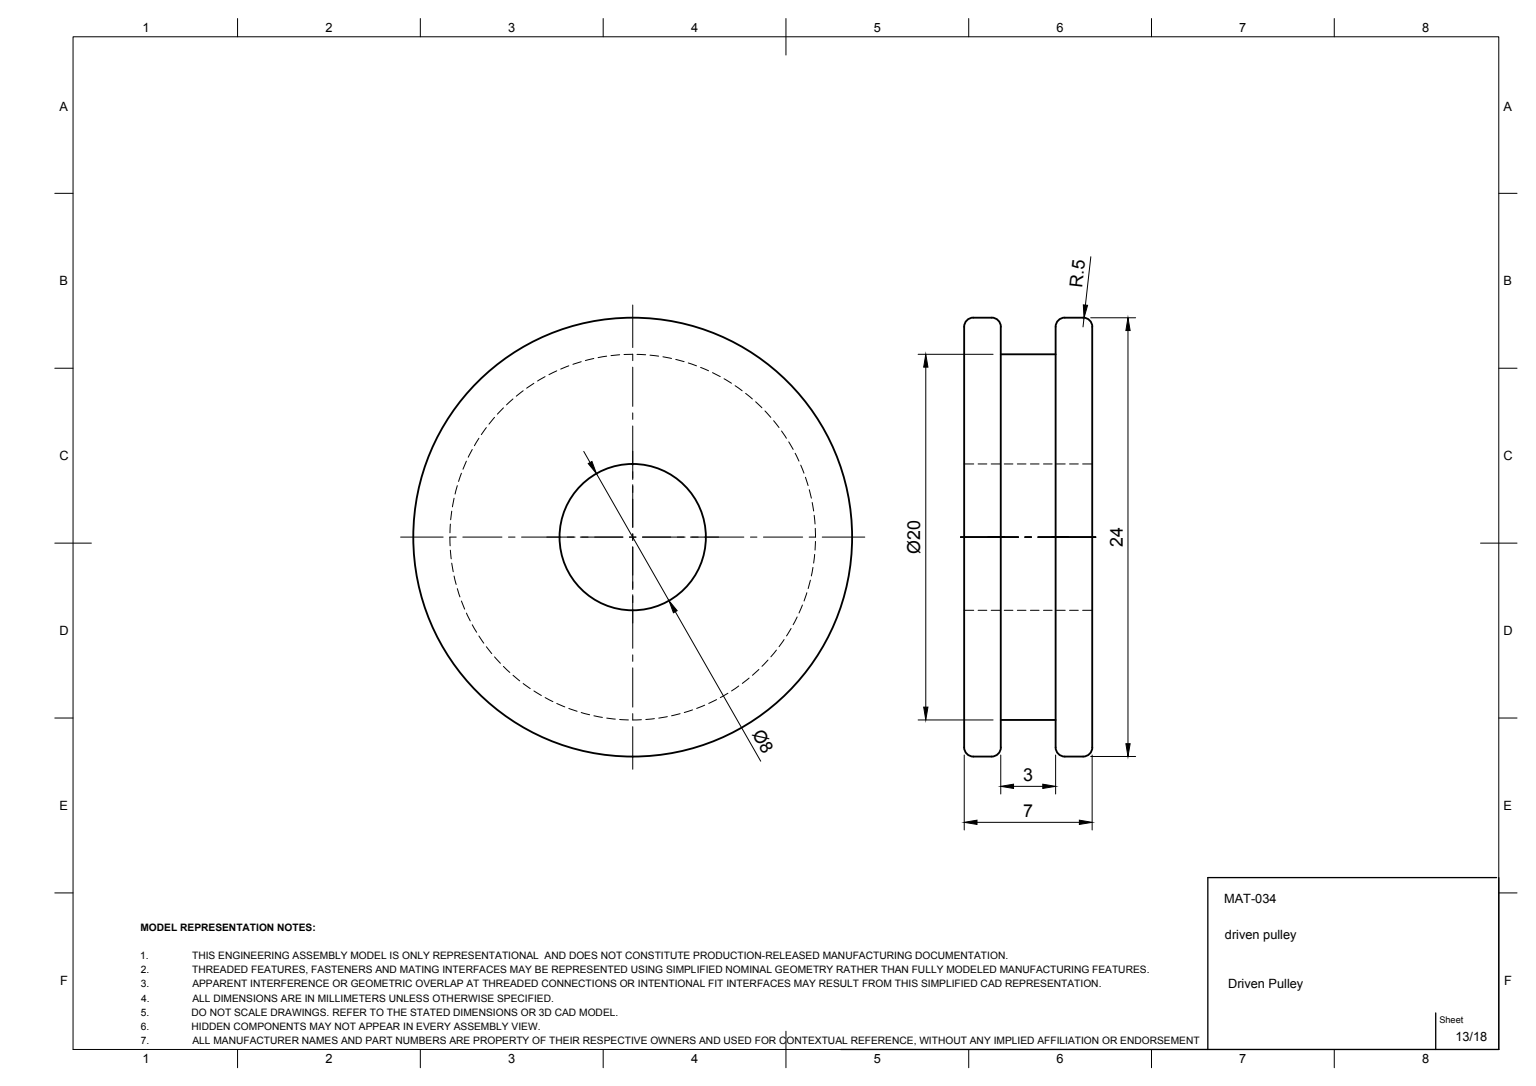
ISO-10303-21;
HEADER;
/* Generated by software containing ST-Developer
 * from STEP Tools, Inc. (www.steptools.com) 
 */

FILE_DESCRIPTION(
/* description */ ('STEP AP214'),
/* implementation_level */ '2;1');

FILE_NAME(
/* name */ 'Driven Pulley.step',
/* time_stamp */ '2026-11-14T09:24:36-08:00',
/* author */ (''),
/* organization */ (''),
/* preprocessor_version */ 'ST-DEVELOPER v20.2',
/* originating_system */ 'Autodesk Translation Framework v15.17.0.0',
/* authorisation */ '');

FILE_SCHEMA (('AUTOMOTIVE_DESIGN { 1 0 10303 214 3 1 1 }'));
ENDSEC;

DATA;
#10=MECHANICAL_DESIGN_GEOMETRIC_PRESENTATION_REPRESENTATION('',(#209),#18867);
#150=TOROIDAL_SURFACE('',#11551,11.5,0.5);
#151=TOROIDAL_SURFACE('',#11555,11.5,0.5);
#152=TOROIDAL_SURFACE('',#11560,11.5,0.5);
#153=TOROIDAL_SURFACE('',#11564,11.5,0.5);
#177=SHAPE_REPRESENTATION_RELATIONSHIP('SRR','None',#18941,#193);
#193=ADVANCED_BREP_SHAPE_REPRESENTATION('',(#233),#18857);
#209=STYLED_ITEM('',(#19027),#233);
#233=MANIFOLD_SOLID_BREP('Body1',#10964);
#323=FACE_BOUND('',#1619,.T.);
#324=FACE_BOUND('',#1621,.T.);
#325=FACE_BOUND('',#1623,.T.);
#326=FACE_BOUND('',#1625,.T.);
#519=PLANE('',#11574);
#520=PLANE('',#11575);
#521=PLANE('',#11576);
#522=PLANE('',#11577);
#942=FACE_OUTER_BOUND('',#1610,.T.);
#943=FACE_OUTER_BOUND('',#1611,.T.);
#944=FACE_OUTER_BOUND('',#1612,.T.);
#945=FACE_OUTER_BOUND('',#1613,.T.);
#946=FACE_OUTER_BOUND('',#1614,.T.);
#947=FACE_OUTER_BOUND('',#1615,.T.);
#948=FACE_OUTER_BOUND('',#1616,.T.);
#949=FACE_OUTER_BOUND('',#1617,.T.);
#950=FACE_OUTER_BOUND('',#1618,.T.);
#951=FACE_OUTER_BOUND('',#1620,.T.);
#952=FACE_OUTER_BOUND('',#1622,.T.);
#953=FACE_OUTER_BOUND('',#1624,.T.);
#1610=EDGE_LOOP('',(#8182,#8183,#8184,#8185));
#1611=EDGE_LOOP('',(#8186,#8187,#8188,#8189));
#1612=EDGE_LOOP('',(#8190,#8191,#8192,#8193,#8194));
#1613=EDGE_LOOP('',(#8195,#8196,#8197,#8198));
#1614=EDGE_LOOP('',(#8199,#8200,#8201,#8202,#8203));
#1615=EDGE_LOOP('',(#8204,#8205,#8206,#8207,#8208));
#1616=EDGE_LOOP('',(#8209,#8210,#8211,#8212));
#1617=EDGE_LOOP('',(#8213,#8214,#8215,#8216,#8217));
#1618=EDGE_LOOP('',(#8218));
#1619=EDGE_LOOP('',(#8219));
#1620=EDGE_LOOP('',(#8220));
#1621=EDGE_LOOP('',(#8221));
#1622=EDGE_LOOP('',(#8222));
#1623=EDGE_LOOP('',(#8223));
#1624=EDGE_LOOP('',(#8224));
#1625=EDGE_LOOP('',(#8225));
#2420=LINE('',#16727,#3434);
#2421=LINE('',#16758,#3435);
#2422=LINE('',#16763,#3436);
#2423=LINE('',#16766,#3437);
#3434=VECTOR('',#13458,4.);
#3435=VECTOR('',#13499,12.);
#3436=VECTOR('',#13504,10.);
#3437=VECTOR('',#13509,12.);
#4235=CIRCLE('',#11549,4.);
#4236=CIRCLE('',#11550,4.);
#4237=CIRCLE('',#11552,12.);
#4238=CIRCLE('',#11553,0.5);
#4239=CIRCLE('',#11554,11.5);
#4240=CIRCLE('',#11556,12.);
#4241=CIRCLE('',#11557,12.);
#4242=CIRCLE('',#11558,0.5);
#4243=CIRCLE('',#11559,11.5);
#4244=CIRCLE('',#11561,12.);
#4245=CIRCLE('',#11562,0.5);
#4246=CIRCLE('',#11563,11.5);
#4247=CIRCLE('',#11565,12.);
#4248=CIRCLE('',#11566,12.);
#4249=CIRCLE('',#11567,0.5);
#4250=CIRCLE('',#11568,11.5);
#4251=CIRCLE('',#11571,10.);
#4252=CIRCLE('',#11572,10.);
#4930=VERTEX_POINT('',#16724);
#4931=VERTEX_POINT('',#16726);
#4932=VERTEX_POINT('',#16730);
#4933=VERTEX_POINT('',#16732);
#4934=VERTEX_POINT('',#16736);
#4935=VERTEX_POINT('',#16737);
#4936=VERTEX_POINT('',#16740);
#4937=VERTEX_POINT('',#16744);
#4938=VERTEX_POINT('',#16746);
#4939=VERTEX_POINT('',#16750);
#4940=VERTEX_POINT('',#16751);
#4941=VERTEX_POINT('',#16754);
#4942=VERTEX_POINT('',#16760);
#4943=VERTEX_POINT('',#16762);
#6124=EDGE_CURVE('',#4930,#4930,#4235,.T.);
#6125=EDGE_CURVE('',#4930,#4931,#2420,.T.);
#6126=EDGE_CURVE('',#4931,#4931,#4236,.T.);
#6127=EDGE_CURVE('',#4932,#4932,#4237,.T.);
#6128=EDGE_CURVE('',#4932,#4933,#4238,.T.);
#6129=EDGE_CURVE('',#4933,#4933,#4239,.T.);
#6130=EDGE_CURVE('',#4934,#4935,#4240,.T.);
#6131=EDGE_CURVE('',#4935,#4934,#4241,.T.);
#6132=EDGE_CURVE('',#4935,#4936,#4242,.T.);
#6133=EDGE_CURVE('',#4936,#4936,#4243,.T.);
#6134=EDGE_CURVE('',#4937,#4937,#4244,.T.);
#6135=EDGE_CURVE('',#4937,#4938,#4245,.T.);
#6136=EDGE_CURVE('',#4938,#4938,#4246,.T.);
#6137=EDGE_CURVE('',#4939,#4940,#4247,.T.);
#6138=EDGE_CURVE('',#4940,#4939,#4248,.T.);
#6139=EDGE_CURVE('',#4940,#4941,#4249,.T.);
#6140=EDGE_CURVE('',#4941,#4941,#4250,.T.);
#6141=EDGE_CURVE('',#4934,#4932,#2421,.T.);
#6142=EDGE_CURVE('',#4942,#4942,#4251,.T.);
#6143=EDGE_CURVE('',#4942,#4943,#2422,.T.);
#6144=EDGE_CURVE('',#4943,#4943,#4252,.T.);
#6145=EDGE_CURVE('',#4939,#4937,#2423,.T.);
#8182=ORIENTED_EDGE('',*,*,#6124,.F.);
#8183=ORIENTED_EDGE('',*,*,#6125,.T.);
#8184=ORIENTED_EDGE('',*,*,#6126,.T.);
#8185=ORIENTED_EDGE('',*,*,#6125,.F.);
#8186=ORIENTED_EDGE('',*,*,#6127,.F.);
#8187=ORIENTED_EDGE('',*,*,#6128,.T.);
#8188=ORIENTED_EDGE('',*,*,#6129,.F.);
#8189=ORIENTED_EDGE('',*,*,#6128,.F.);
#8190=ORIENTED_EDGE('',*,*,#6130,.F.);
#8191=ORIENTED_EDGE('',*,*,#6131,.F.);
#8192=ORIENTED_EDGE('',*,*,#6132,.T.);
#8193=ORIENTED_EDGE('',*,*,#6133,.F.);
#8194=ORIENTED_EDGE('',*,*,#6132,.F.);
#8195=ORIENTED_EDGE('',*,*,#6134,.F.);
#8196=ORIENTED_EDGE('',*,*,#6135,.T.);
#8197=ORIENTED_EDGE('',*,*,#6136,.F.);
#8198=ORIENTED_EDGE('',*,*,#6135,.F.);
#8199=ORIENTED_EDGE('',*,*,#6137,.F.);
#8200=ORIENTED_EDGE('',*,*,#6138,.F.);
#8201=ORIENTED_EDGE('',*,*,#6139,.T.);
#8202=ORIENTED_EDGE('',*,*,#6140,.F.);
#8203=ORIENTED_EDGE('',*,*,#6139,.F.);
#8204=ORIENTED_EDGE('',*,*,#6130,.T.);
#8205=ORIENTED_EDGE('',*,*,#6131,.T.);
#8206=ORIENTED_EDGE('',*,*,#6141,.T.);
#8207=ORIENTED_EDGE('',*,*,#6127,.T.);
#8208=ORIENTED_EDGE('',*,*,#6141,.F.);
#8209=ORIENTED_EDGE('',*,*,#6142,.F.);
#8210=ORIENTED_EDGE('',*,*,#6143,.T.);
#8211=ORIENTED_EDGE('',*,*,#6144,.T.);
#8212=ORIENTED_EDGE('',*,*,#6143,.F.);
#8213=ORIENTED_EDGE('',*,*,#6137,.T.);
#8214=ORIENTED_EDGE('',*,*,#6138,.T.);
#8215=ORIENTED_EDGE('',*,*,#6145,.T.);
#8216=ORIENTED_EDGE('',*,*,#6134,.T.);
#8217=ORIENTED_EDGE('',*,*,#6145,.F.);
#8218=ORIENTED_EDGE('',*,*,#6129,.T.);
#8219=ORIENTED_EDGE('',*,*,#6124,.T.);
#8220=ORIENTED_EDGE('',*,*,#6140,.T.);
#8221=ORIENTED_EDGE('',*,*,#6126,.F.);
#8222=ORIENTED_EDGE('',*,*,#6136,.T.);
#8223=ORIENTED_EDGE('',*,*,#6142,.T.);
#8224=ORIENTED_EDGE('',*,*,#6133,.T.);
#8225=ORIENTED_EDGE('',*,*,#6144,.F.);
#10225=CYLINDRICAL_SURFACE('',#11548,4.);
#10226=CYLINDRICAL_SURFACE('',#11569,12.);
#10227=CYLINDRICAL_SURFACE('',#11570,10.);
#10228=CYLINDRICAL_SURFACE('',#11573,12.);
#10579=ADVANCED_FACE('',(#942),#10225,.F.);
#10580=ADVANCED_FACE('',(#943),#150,.T.);
#10581=ADVANCED_FACE('',(#944),#151,.T.);
#10582=ADVANCED_FACE('',(#945),#152,.T.);
#10583=ADVANCED_FACE('',(#946),#153,.T.);
#10584=ADVANCED_FACE('',(#947),#10226,.T.);
#10585=ADVANCED_FACE('',(#948),#10227,.T.);
#10586=ADVANCED_FACE('',(#949),#10228,.T.);
#10587=ADVANCED_FACE('',(#950,#323),#519,.F.);
#10588=ADVANCED_FACE('',(#951,#324),#520,.F.);
#10589=ADVANCED_FACE('',(#952,#325),#521,.F.);
#10590=ADVANCED_FACE('',(#953,#326),#522,.F.);
#10964=CLOSED_SHELL('',(#10579,#10580,#10581,#10582,#10583,#10584,#10585,
#10586,#10587,#10588,#10589,#10590));
#11547=AXIS2_PLACEMENT_3D('',#16722,#13452,#13453);
#11548=AXIS2_PLACEMENT_3D('',#16723,#13454,#13455);
#11549=AXIS2_PLACEMENT_3D('',#16725,#13456,#13457);
#11550=AXIS2_PLACEMENT_3D('',#16728,#13459,#13460);
#11551=AXIS2_PLACEMENT_3D('',#16729,#13461,#13462);
#11552=AXIS2_PLACEMENT_3D('',#16731,#13463,#13464);
#11553=AXIS2_PLACEMENT_3D('',#16733,#13465,#13466);
#11554=AXIS2_PLACEMENT_3D('',#16734,#13467,#13468);
#11555=AXIS2_PLACEMENT_3D('',#16735,#13469,#13470);
#11556=AXIS2_PLACEMENT_3D('',#16738,#13471,#13472);
#11557=AXIS2_PLACEMENT_3D('',#16739,#13473,#13474);
#11558=AXIS2_PLACEMENT_3D('',#16741,#13475,#13476);
#11559=AXIS2_PLACEMENT_3D('',#16742,#13477,#13478);
#11560=AXIS2_PLACEMENT_3D('',#16743,#13479,#13480);
#11561=AXIS2_PLACEMENT_3D('',#16745,#13481,#13482);
#11562=AXIS2_PLACEMENT_3D('',#16747,#13483,#13484);
#11563=AXIS2_PLACEMENT_3D('',#16748,#13485,#13486);
#11564=AXIS2_PLACEMENT_3D('',#16749,#13487,#13488);
#11565=AXIS2_PLACEMENT_3D('',#16752,#13489,#13490);
#11566=AXIS2_PLACEMENT_3D('',#16753,#13491,#13492);
#11567=AXIS2_PLACEMENT_3D('',#16755,#13493,#13494);
#11568=AXIS2_PLACEMENT_3D('',#16756,#13495,#13496);
#11569=AXIS2_PLACEMENT_3D('',#16757,#13497,#13498);
#11570=AXIS2_PLACEMENT_3D('',#16759,#13500,#13501);
#11571=AXIS2_PLACEMENT_3D('',#16761,#13502,#13503);
#11572=AXIS2_PLACEMENT_3D('',#16764,#13505,#13506);
#11573=AXIS2_PLACEMENT_3D('',#16765,#13507,#13508);
#11574=AXIS2_PLACEMENT_3D('',#16767,#13510,#13511);
#11575=AXIS2_PLACEMENT_3D('',#16768,#13512,#13513);
#11576=AXIS2_PLACEMENT_3D('',#16769,#13514,#13515);
#11577=AXIS2_PLACEMENT_3D('',#16770,#13516,#13517);
#13452=DIRECTION('axis',(0.,0.,1.));
#13453=DIRECTION('refdir',(1.,0.,0.));
#13454=DIRECTION('center_axis',(-1.,0.,0.));
#13455=DIRECTION('ref_axis',(0.,0.,1.));
#13456=DIRECTION('center_axis',(-1.,0.,0.));
#13457=DIRECTION('ref_axis',(0.,0.,1.));
#13458=DIRECTION('',(-1.,0.,0.));
#13459=DIRECTION('center_axis',(-1.,0.,0.));
#13460=DIRECTION('ref_axis',(0.,0.,1.));
#13461=DIRECTION('center_axis',(-1.,0.,0.));
#13462=DIRECTION('ref_axis',(0.,0.,1.));
#13463=DIRECTION('center_axis',(-1.,0.,0.));
#13464=DIRECTION('ref_axis',(0.,0.,1.));
#13465=DIRECTION('center_axis',(0.,-1.,1.22464679914735E-16));
#13466=DIRECTION('ref_axis',(0.,-1.22464679914735E-16,-1.));
#13467=DIRECTION('center_axis',(1.,0.,0.));
#13468=DIRECTION('ref_axis',(0.,0.,1.));
#13469=DIRECTION('center_axis',(1.,0.,0.));
#13470=DIRECTION('ref_axis',(0.,0.,-1.));
#13471=DIRECTION('center_axis',(1.,0.,0.));
#13472=DIRECTION('ref_axis',(0.,0.,-1.));
#13473=DIRECTION('center_axis',(1.,0.,0.));
#13474=DIRECTION('ref_axis',(0.,0.,-1.));
#13475=DIRECTION('center_axis',(0.,-1.,-1.22464679914735E-16));
#13476=DIRECTION('ref_axis',(0.,-1.22464679914735E-16,1.));
#13477=DIRECTION('center_axis',(-1.,0.,0.));
#13478=DIRECTION('ref_axis',(0.,0.,-1.));
#13479=DIRECTION('center_axis',(-1.,0.,0.));
#13480=DIRECTION('ref_axis',(0.,0.,1.));
#13481=DIRECTION('center_axis',(-1.,0.,0.));
#13482=DIRECTION('ref_axis',(0.,0.,1.));
#13483=DIRECTION('center_axis',(0.,-1.,1.22464679914735E-16));
#13484=DIRECTION('ref_axis',(0.,-1.22464679914735E-16,-1.));
#13485=DIRECTION('center_axis',(1.,0.,0.));
#13486=DIRECTION('ref_axis',(0.,0.,1.));
#13487=DIRECTION('center_axis',(1.,0.,0.));
#13488=DIRECTION('ref_axis',(0.,0.,-1.));
#13489=DIRECTION('center_axis',(1.,0.,0.));
#13490=DIRECTION('ref_axis',(0.,0.,-1.));
#13491=DIRECTION('center_axis',(1.,0.,0.));
#13492=DIRECTION('ref_axis',(0.,0.,-1.));
#13493=DIRECTION('center_axis',(0.,-1.,-1.22464679914735E-16));
#13494=DIRECTION('ref_axis',(0.,-1.22464679914735E-16,1.));
#13495=DIRECTION('center_axis',(-1.,0.,0.));
#13496=DIRECTION('ref_axis',(0.,0.,-1.));
#13497=DIRECTION('center_axis',(-1.,0.,0.));
#13498=DIRECTION('ref_axis',(0.,0.,1.));
#13499=DIRECTION('',(1.,0.,0.));
#13500=DIRECTION('center_axis',(-1.,0.,0.));
#13501=DIRECTION('ref_axis',(0.,0.,1.));
#13502=DIRECTION('center_axis',(-1.,0.,0.));
#13503=DIRECTION('ref_axis',(0.,0.,1.));
#13504=DIRECTION('',(1.,0.,0.));
#13505=DIRECTION('center_axis',(-1.,0.,0.));
#13506=DIRECTION('ref_axis',(0.,0.,1.));
#13507=DIRECTION('center_axis',(-1.,0.,0.));
#13508=DIRECTION('ref_axis',(0.,0.,1.));
#13509=DIRECTION('',(1.,0.,0.));
#13510=DIRECTION('center_axis',(-1.,0.,0.));
#13511=DIRECTION('ref_axis',(0.,0.,1.));
#13512=DIRECTION('center_axis',(1.,0.,0.));
#13513=DIRECTION('ref_axis',(0.,0.,-1.));
#13514=DIRECTION('center_axis',(-1.,0.,0.));
#13515=DIRECTION('ref_axis',(0.,0.,1.));
#13516=DIRECTION('center_axis',(1.,0.,0.));
#13517=DIRECTION('ref_axis',(0.,0.,-1.));
#16722=CARTESIAN_POINT('',(0.,0.,0.));
#16723=CARTESIAN_POINT('Origin',(3.5,0.,0.));
#16724=CARTESIAN_POINT('',(3.5,-4.89858719658941E-16,-4.));
#16725=CARTESIAN_POINT('Origin',(3.5,0.,0.));
#16726=CARTESIAN_POINT('',(-3.5,-4.89858719658941E-16,-4.));
#16727=CARTESIAN_POINT('',(3.5,-4.89858719658941E-16,-4.));
#16728=CARTESIAN_POINT('Origin',(-3.5,0.,0.));
#16729=CARTESIAN_POINT('Origin',(3.,0.,0.));
#16730=CARTESIAN_POINT('',(3.,-1.46957615897682E-15,-12.));
#16731=CARTESIAN_POINT('Origin',(3.,0.,0.));
#16732=CARTESIAN_POINT('',(3.5,-1.40834381901946E-15,-11.5));
#16733=CARTESIAN_POINT('Origin',(3.,-1.40834381901946E-15,-11.5));
#16734=CARTESIAN_POINT('Origin',(3.5,0.,0.));
#16735=CARTESIAN_POINT('Origin',(2.,0.,0.));
#16736=CARTESIAN_POINT('',(2.,1.46957615897682E-15,-12.));
#16737=CARTESIAN_POINT('',(2.,-1.46957615897682E-15,12.));
#16738=CARTESIAN_POINT('Origin',(2.,0.,0.));
#16739=CARTESIAN_POINT('Origin',(2.,0.,0.));
#16740=CARTESIAN_POINT('',(1.5,-1.40834381901946E-15,11.5));
#16741=CARTESIAN_POINT('Origin',(2.,-1.40834381901946E-15,11.5));
#16742=CARTESIAN_POINT('Origin',(1.5,0.,0.));
#16743=CARTESIAN_POINT('Origin',(-2.,0.,0.));
#16744=CARTESIAN_POINT('',(-2.,-1.46957615897682E-15,-12.));
#16745=CARTESIAN_POINT('Origin',(-2.,0.,0.));
#16746=CARTESIAN_POINT('',(-1.5,-1.40834381901946E-15,-11.5));
#16747=CARTESIAN_POINT('Origin',(-2.,-1.40834381901946E-15,-11.5));
#16748=CARTESIAN_POINT('Origin',(-1.5,0.,0.));
#16749=CARTESIAN_POINT('Origin',(-3.,0.,0.));
#16750=CARTESIAN_POINT('',(-3.,1.46957615897682E-15,-12.));
#16751=CARTESIAN_POINT('',(-3.,-1.46957615897682E-15,12.));
#16752=CARTESIAN_POINT('Origin',(-3.,0.,0.));
#16753=CARTESIAN_POINT('Origin',(-3.,0.,0.));
#16754=CARTESIAN_POINT('',(-3.5,-1.40834381901946E-15,11.5));
#16755=CARTESIAN_POINT('Origin',(-3.,-1.40834381901946E-15,11.5));
#16756=CARTESIAN_POINT('Origin',(-3.5,0.,0.));
#16757=CARTESIAN_POINT('Origin',(-3.5,0.,0.));
#16758=CARTESIAN_POINT('',(-3.5,-1.46957615897682E-15,-12.));
#16759=CARTESIAN_POINT('Origin',(-3.5,0.,0.));
#16760=CARTESIAN_POINT('',(-1.5,-1.22464679914735E-15,-10.));
#16761=CARTESIAN_POINT('Origin',(-1.5,0.,0.));
#16762=CARTESIAN_POINT('',(1.5,-1.22464679914735E-15,-10.));
#16763=CARTESIAN_POINT('',(-3.5,-1.22464679914735E-15,-10.));
#16764=CARTESIAN_POINT('Origin',(1.5,0.,0.));
#16765=CARTESIAN_POINT('Origin',(-3.5,0.,0.));
#16766=CARTESIAN_POINT('',(-3.5,-1.46957615897682E-15,-12.));
#16767=CARTESIAN_POINT('Origin',(3.5,12.,0.));
#16768=CARTESIAN_POINT('Origin',(-3.5,0.,0.));
#16769=CARTESIAN_POINT('Origin',(-1.5,12.,0.));
#16770=CARTESIAN_POINT('Origin',(1.5,10.,0.));
#18839=UNCERTAINTY_MEASURE_WITH_UNIT(LENGTH_MEASURE(0.01),#18868,
'DISTANCE_ACCURACY_VALUE',
'Maximum model space distance between geometric entities at asserted c
onnectivities');
#18849=UNCERTAINTY_MEASURE_WITH_UNIT(LENGTH_MEASURE(0.01),#18868,
'DISTANCE_ACCURACY_VALUE',
'Maximum model space distance between geometric entities at asserted c
onnectivities');
#18857=(
GEOMETRIC_REPRESENTATION_CONTEXT(3)
GLOBAL_UNCERTAINTY_ASSIGNED_CONTEXT((#18839))
GLOBAL_UNIT_ASSIGNED_CONTEXT((#18868,#18870,#18871))
REPRESENTATION_CONTEXT('','3D')
);
#18867=(
GEOMETRIC_REPRESENTATION_CONTEXT(3)
GLOBAL_UNCERTAINTY_ASSIGNED_CONTEXT((#18849))
GLOBAL_UNIT_ASSIGNED_CONTEXT((#18868,#18870,#18871))
REPRESENTATION_CONTEXT('','3D')
);
#18868=(
LENGTH_UNIT()
NAMED_UNIT(*)
SI_UNIT(.MILLI.,.METRE.)
);
#18870=(
NAMED_UNIT(*)
PLANE_ANGLE_UNIT()
SI_UNIT($,.RADIAN.)
);
#18871=(
NAMED_UNIT(*)
SI_UNIT($,.STERADIAN.)
SOLID_ANGLE_UNIT()
);
#18879=SHAPE_DEFINITION_REPRESENTATION(#18896,#18941);
#18896=PRODUCT_DEFINITION_SHAPE('',$,#18959);
#18941=SHAPE_REPRESENTATION('',(#11547),#18857);
#18951=PRODUCT_DEFINITION_CONTEXT('part definition',#19004,'design');
#18959=PRODUCT_DEFINITION('driven pulley','Driven Pulley',#18976,#18951);
#18976=PRODUCT_DEFINITION_FORMATION('',$,#19013);
#19004=APPLICATION_CONTEXT(
'Core Data for Automotive Mechanical Design Process');
#19005=PRODUCT_CONTEXT('part definition',#19004,'mechanical');
#19013=PRODUCT('driven pulley','Driven Pulley',$,(#19005));
#19027=PRESENTATION_STYLE_ASSIGNMENT((#19033));
#19033=SURFACE_STYLE_USAGE(.BOTH.,#19039);
#19039=SURFACE_SIDE_STYLE('',(#19045));
#19045=SURFACE_STYLE_FILL_AREA(#19051);
#19051=FILL_AREA_STYLE('Opaque(122,133,145)',(#19057));
#19057=FILL_AREA_STYLE_COLOUR('Opaque(122,133,145)',#19063);
#19063=COLOUR_RGB('Opaque(122,133,145)',0.47843137254902,0.52156862745098,
0.568627450980392);
ENDSEC;
END-ISO-10303-21;
